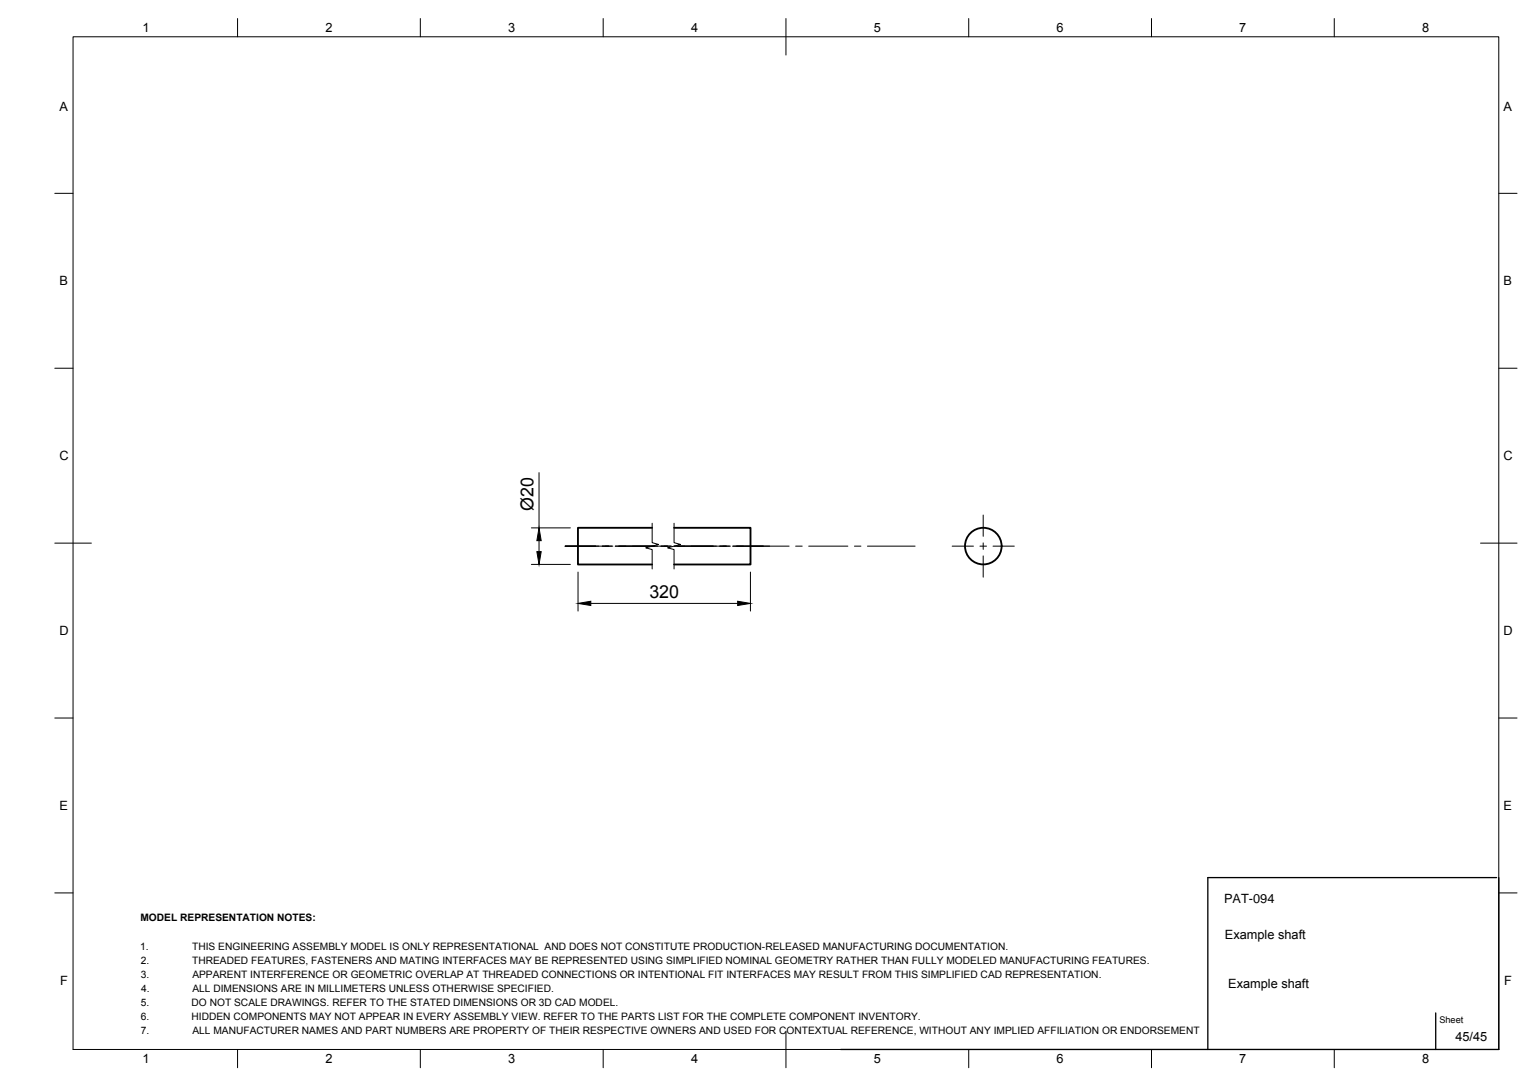
ISO-10303-21;
HEADER;
/* Generated by software containing ST-Developer
 * from STEP Tools, Inc. (www.steptools.com) 
 */

FILE_DESCRIPTION(
/* description */ ('Shaft runout checking stand'),
/* implementation_level */ '2;1');

FILE_NAME(
/* name */ 'Example shaft.step',
/* time_stamp */ '2026-11-02T21:12:33-08:00',
/* author */ (''),
/* organization */ (''),
/* preprocessor_version */ 'ST-DEVELOPER v20.2',
/* originating_system */ 'Autodesk Translation Framework v15.17.0.0',
/* authorisation */ '');

FILE_SCHEMA (('AUTOMOTIVE_DESIGN { 1 0 10303 214 3 1 1 }'));
ENDSEC;

DATA;
#10=MECHANICAL_DESIGN_GEOMETRIC_PRESENTATION_REPRESENTATION('',(#497),#11748);
#411=SHAPE_REPRESENTATION_RELATIONSHIP('SRR','None',#11961,#454);
#454=ADVANCED_BREP_SHAPE_REPRESENTATION('',(#545),#11737);
#497=STYLED_ITEM('',(#12170),#545);
#545=MANIFOLD_SOLID_BREP('Body1',#6243);
#852=CIRCLE('',#7315,1.);
#853=CIRCLE('',#7316,1.);
#1019=CYLINDRICAL_SURFACE('',#7314,1.);
#1340=FACE_OUTER_BOUND('',#1804,.T.);
#1341=FACE_OUTER_BOUND('',#1805,.T.);
#1342=FACE_OUTER_BOUND('',#1806,.T.);
#1804=EDGE_LOOP('',(#5350,#5351,#5352,#5353));
#1805=EDGE_LOOP('',(#5354));
#1806=EDGE_LOOP('',(#5355));
#2329=LINE('',#11004,#2796);
#2796=VECTOR('',#9100,1.);
#3236=VERTEX_POINT('',#11001);
#3237=VERTEX_POINT('',#11003);
#3961=EDGE_CURVE('',#3236,#3236,#852,.T.);
#3962=EDGE_CURVE('',#3236,#3237,#2329,.T.);
#3963=EDGE_CURVE('',#3237,#3237,#853,.T.);
#5350=ORIENTED_EDGE('',*,*,#3961,.F.);
#5351=ORIENTED_EDGE('',*,*,#3962,.T.);
#5352=ORIENTED_EDGE('',*,*,#3963,.T.);
#5353=ORIENTED_EDGE('',*,*,#3962,.F.);
#5354=ORIENTED_EDGE('',*,*,#3961,.T.);
#5355=ORIENTED_EDGE('',*,*,#3963,.F.);
#5813=PLANE('',#7317);
#5814=PLANE('',#7318);
#6140=ADVANCED_FACE('',(#1340),#1019,.T.);
#6141=ADVANCED_FACE('',(#1341),#5813,.T.);
#6142=ADVANCED_FACE('',(#1342),#5814,.F.);
#6243=CLOSED_SHELL('',(#6140,#6141,#6142));
#7313=AXIS2_PLACEMENT_3D('',#10999,#9094,#9095);
#7314=AXIS2_PLACEMENT_3D('',#11000,#9096,#9097);
#7315=AXIS2_PLACEMENT_3D('',#11002,#9098,#9099);
#7316=AXIS2_PLACEMENT_3D('',#11005,#9101,#9102);
#7317=AXIS2_PLACEMENT_3D('',#11006,#9103,#9104);
#7318=AXIS2_PLACEMENT_3D('',#11007,#9105,#9106);
#9094=DIRECTION('axis',(0.,0.,1.));
#9095=DIRECTION('refdir',(1.,0.,0.));
#9096=DIRECTION('center_axis',(0.,1.,0.));
#9097=DIRECTION('ref_axis',(1.,0.,0.));
#9098=DIRECTION('center_axis',(0.,1.,0.));
#9099=DIRECTION('ref_axis',(1.,0.,0.));
#9100=DIRECTION('',(0.,-1.,0.));
#9101=DIRECTION('center_axis',(0.,1.,0.));
#9102=DIRECTION('ref_axis',(1.,0.,0.));
#9103=DIRECTION('center_axis',(0.,1.,0.));
#9104=DIRECTION('ref_axis',(1.,0.,0.));
#9105=DIRECTION('center_axis',(0.,1.,0.));
#9106=DIRECTION('ref_axis',(1.,0.,0.));
#10999=CARTESIAN_POINT('',(0.,0.,0.));
#11000=CARTESIAN_POINT('Origin',(0.,-16.,6.95959179422654));
#11001=CARTESIAN_POINT('',(-1.,16.,6.95959179422654));
#11002=CARTESIAN_POINT('Origin',(0.,16.,6.95959179422654));
#11003=CARTESIAN_POINT('',(-1.,-16.,6.95959179422654));
#11004=CARTESIAN_POINT('',(-1.,-16.,6.95959179422654));
#11005=CARTESIAN_POINT('Origin',(0.,-16.,6.95959179422654));
#11006=CARTESIAN_POINT('Origin',(0.,16.,6.95959179422654));
#11007=CARTESIAN_POINT('Origin',(0.,-16.,6.95959179422654));
#11688=UNCERTAINTY_MEASURE_WITH_UNIT(LENGTH_MEASURE(0.001),#11749,
'DISTANCE_ACCURACY_VALUE',
'Maximum model space distance between geometric entities at asserted c
onnectivities');
#11699=UNCERTAINTY_MEASURE_WITH_UNIT(LENGTH_MEASURE(0.001),#11749,
'DISTANCE_ACCURACY_VALUE',
'Maximum model space distance between geometric entities at asserted c
onnectivities');
#11737=(
GEOMETRIC_REPRESENTATION_CONTEXT(3)
GLOBAL_UNCERTAINTY_ASSIGNED_CONTEXT((#11688))
GLOBAL_UNIT_ASSIGNED_CONTEXT((#11749,#11751,#11752))
REPRESENTATION_CONTEXT('','3D')
);
#11748=(
GEOMETRIC_REPRESENTATION_CONTEXT(3)
GLOBAL_UNCERTAINTY_ASSIGNED_CONTEXT((#11699))
GLOBAL_UNIT_ASSIGNED_CONTEXT((#11749,#11751,#11752))
REPRESENTATION_CONTEXT('','3D')
);
#11749=(
LENGTH_UNIT()
NAMED_UNIT(*)
SI_UNIT(.CENTI.,.METRE.)
);
#11751=(
NAMED_UNIT(*)
PLANE_ANGLE_UNIT()
SI_UNIT($,.RADIAN.)
);
#11752=(
NAMED_UNIT(*)
SI_UNIT($,.STERADIAN.)
SOLID_ANGLE_UNIT()
);
#11790=SHAPE_DEFINITION_REPRESENTATION(#11897,#11961);
#11897=PRODUCT_DEFINITION_SHAPE('',$,#12010);
#11961=SHAPE_REPRESENTATION('',(#7313),#11737);
#11972=PRODUCT_DEFINITION_CONTEXT('part definition',#12118,'design');
#12010=PRODUCT_DEFINITION('Example shaft_1','Example shaft',#12058,#11972);
#12058=PRODUCT_DEFINITION_FORMATION('',$,#12157);
#12118=APPLICATION_CONTEXT(
'Core Data for Automotive Mechanical Design Process');
#12119=PRODUCT_CONTEXT('part definition',#12118,'mechanical');
#12157=PRODUCT('Example shaft_1','Example shaft','Example shaft',(#12119));
#12170=PRESENTATION_STYLE_ASSIGNMENT((#12175));
#12175=SURFACE_STYLE_USAGE(.BOTH.,#12180);
#12180=SURFACE_SIDE_STYLE('',(#12185));
#12185=SURFACE_STYLE_FILL_AREA(#12190);
#12190=FILL_AREA_STYLE('CAD Library Painted - Steel gray',(#12195));
#12195=FILL_AREA_STYLE_COLOUR('CAD Library Painted - Steel gray',#12200);
#12200=COLOUR_RGB('CAD Library Painted - Steel gray',0.592156862745098,
0.631372549019608,0.67843137254902);
ENDSEC;
END-ISO-10303-21;
